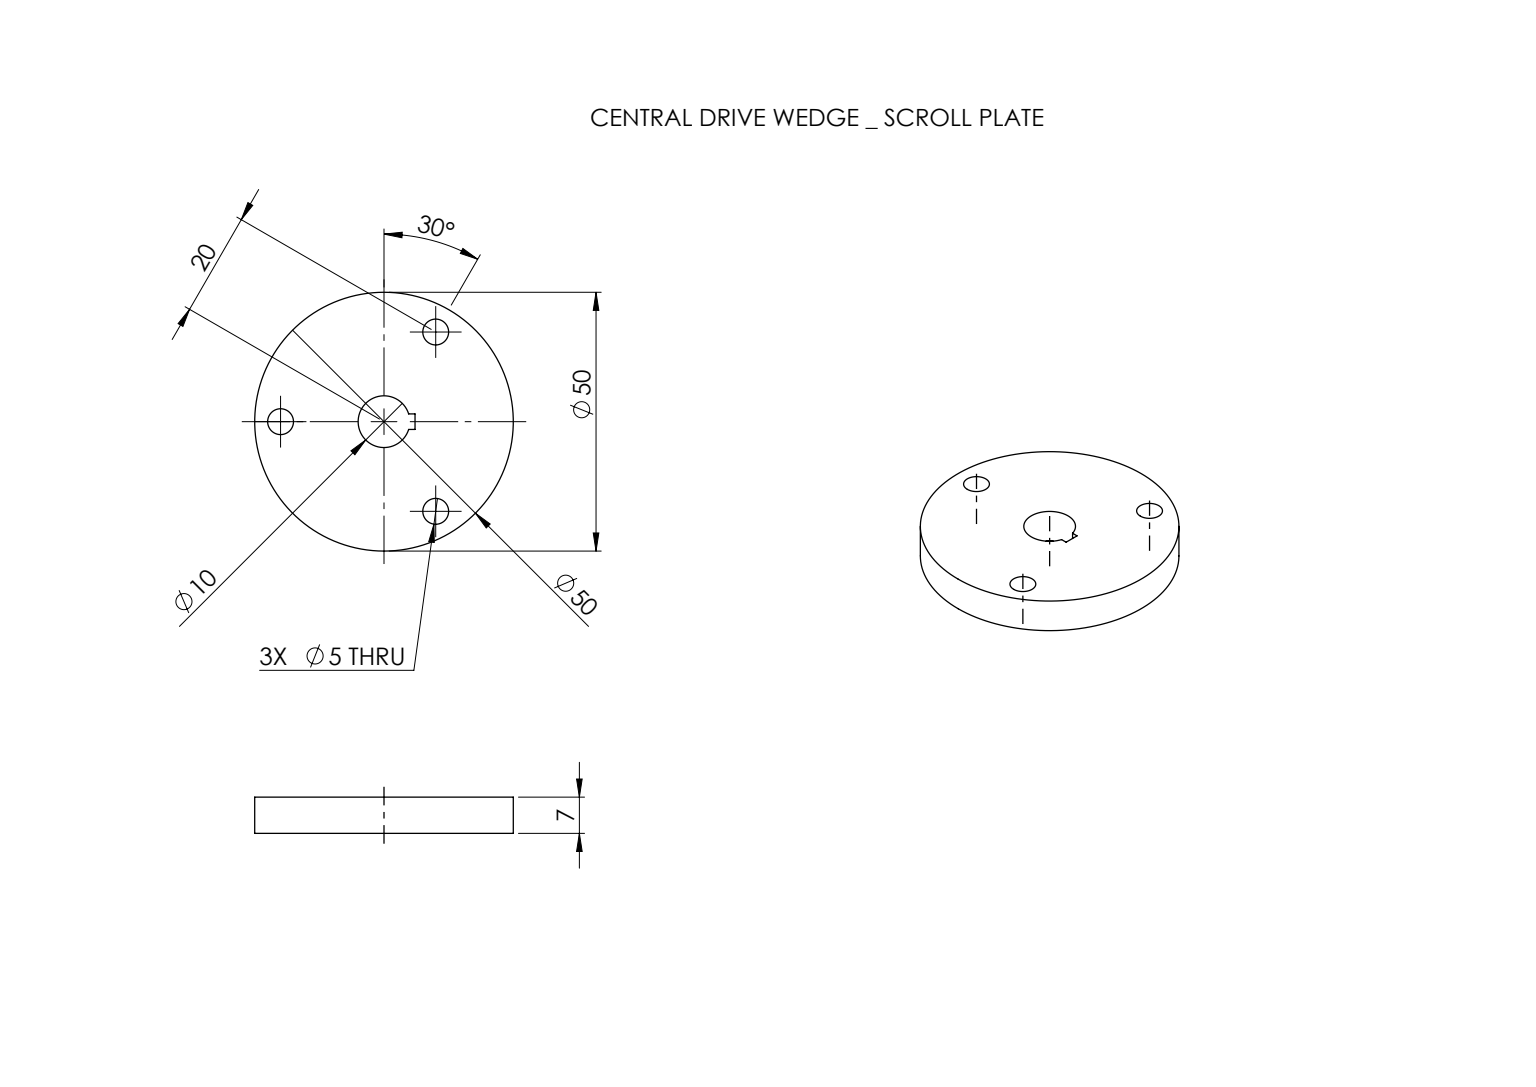
ISO-10303-21;
HEADER;
FILE_DESCRIPTION (('STEP AP214'),
    '1' );
FILE_NAME ('Central Drive Wedge _ Scroll Plate.step',
    '2026-10-08T13:56:24',
    ( '' ),
    ( '' ),
    'SwSTEP 2.0',
    'SolidWorks 2026',
    '' );
FILE_SCHEMA (( 'AUTOMOTIVE_DESIGN' ));
ENDSEC;

DATA;
#7=CARTESIAN_POINT ( 'NONE',  ( -19.99999999999956657, -20.00000000000000000, 2.500000000000877520 ) ) ;
#32=SURFACE_STYLE_USAGE ( .BOTH. , #3487 ) ;
#36=EDGE_CURVE ( 'NONE', #5349, #13611, #14887, .T. ) ;
#57=AXIS2_PLACEMENT_3D ( 'NONE', #12926, #4133, #15222 ) ;
#85=PLANE ( 'NONE',  #15054 ) ;
#94=PRESENTATION_STYLE_ASSIGNMENT (( #15940 ) ) ;
#166=EDGE_LOOP ( 'NONE', ( #524, #8301 ) ) ;
#170=CARTESIAN_POINT ( 'NONE',  ( -19.99999999999956657, -13.00000000000000178, -2.499999999999120259 ) ) ;
#196=DIRECTION ( 'NONE',  ( 0.000000000000000000, 1.000000000000000000, 0.000000000000000000 ) ) ;
#198=ORIENTED_EDGE ( 'NONE', *, *, #1877, .T. ) ;
#211=AXIS2_PLACEMENT_3D ( 'NONE', #9858, #13319, #2262 ) ;
#223=EDGE_CURVE ( 'NONE', #8492, #2510, #15229, .T. ) ;
#249=ORIENTED_EDGE ( 'NONE', *, *, #671, .F. ) ;
#255=FACE_OUTER_BOUND ( 'NONE', #7312, .T. ) ;
#286=DIRECTION ( 'NONE',  ( -0.000000000000000000, -1.000000000000000000, -0.000000000000000000 ) ) ;
#320=DIRECTION ( 'NONE',  ( 0.000000000000000000, 0.000000000000000000, 1.000000000000000000 ) ) ;
#354=CYLINDRICAL_SURFACE ( 'NONE', #57, 2.500000000000000444 ) ;
#358=CARTESIAN_POINT ( 'NONE',  ( -19.99999999999956657, -20.00000000000000000, 8.786575603324269439E-13 ) ) ;
#370=DIRECTION ( 'NONE',  ( -1.000000000000000000, 0.000000000000000000, -0.000000000000000000 ) ) ;
#437=EDGE_CURVE ( 'NONE', #15006, #14231, #6144, .T. ) ;
#524=ORIENTED_EDGE ( 'NONE', *, *, #6442, .T. ) ;
#527=CARTESIAN_POINT ( 'NONE',  ( 9.999999999999891642, -13.00000000000000178, -17.32050807568883499 ) ) ;
#606=CARTESIAN_POINT ( 'NONE',  ( 3.061616997868383043E-15, -13.00000000000000178, 25.00000000000000000 ) ) ;
#609=PRODUCT ( 'Central Drive Wedge _ Scroll Plate', 'Central Drive Wedge _ Scroll Plate', '', ( #8672 ) ) ;
#629=CARTESIAN_POINT ( 'NONE',  ( 0.000000000000000000, -13.00000000000000178, 0.000000000000000000 ) ) ;
#638=ORIENTED_EDGE ( 'NONE', *, *, #11162, .F. ) ;
#644=AXIS2_PLACEMENT_3D ( 'NONE', #5171, #10099, #12584 ) ;
#669=DIRECTION ( 'NONE',  ( 0.000000000000000000, 0.000000000000000000, 1.000000000000000000 ) ) ;
#671=EDGE_CURVE ( 'NONE', #11646, #7839, #3553, .T. ) ;
#723=APPLICATION_CONTEXT ( 'automotive_design' ) ;
#730=DIRECTION ( 'NONE',  ( 0.000000000000000000, 0.000000000000000000, -1.000000000000000000 ) ) ;
#737=DIRECTION ( 'NONE',  ( -0.000000000000000000, -1.000000000000000000, -0.000000000000000000 ) ) ;
#745=CIRCLE ( 'NONE', #4086, 2.499999999999998668 ) ;
#773=EDGE_LOOP ( 'NONE', ( #6443, #12124, #14926, #9073 ) ) ;
#853=DIRECTION ( 'NONE',  ( 0.000000000000000000, 1.000000000000000000, 0.000000000000000000 ) ) ;
#854=CIRCLE ( 'NONE', #9367, 2.499999999999998668 ) ;
#857=CARTESIAN_POINT ( 'NONE',  ( 4.769696007084728073, -20.00000000000000000, -1.500000000000000000 ) ) ;
#869=VERTEX_POINT ( 'NONE', #9235 ) ;
#918=AXIS2_PLACEMENT_3D ( 'NONE', #15837, #15765, #9600 ) ;
#928=VERTEX_POINT ( 'NONE', #6734 ) ;
#931=ORIENTED_EDGE ( 'NONE', *, *, #3922, .F. ) ;
#935=CARTESIAN_POINT ( 'NONE',  ( 0.000000000000000000, -20.00000000000000000, 0.000000000000000000 ) ) ;
#1000=DIRECTION ( 'NONE',  ( -0.000000000000000000, -1.000000000000000000, -0.000000000000000000 ) ) ;
#1016=LINE ( 'NONE', #4965, #2526 ) ;
#1021=AXIS2_PLACEMENT_3D ( 'NONE', #527, #286, #7723 ) ;
#1047=CARTESIAN_POINT ( 'NONE',  ( 6.000000000000000000, -20.00000000000000000, 1.500000000000000000 ) ) ;
#1069=EDGE_LOOP ( 'NONE', ( #13580, #15469, #3315, #3056 ) ) ;
#1076=ADVANCED_FACE ( 'NONE', ( #7046 ), #10609, .T. ) ;
#1110=CARTESIAN_POINT ( 'NONE',  ( 3.061616997868383043E-15, -20.00000000000000000, 25.00000000000000000 ) ) ;
#1136=CARTESIAN_POINT ( 'NONE',  ( 0.000000000000000000, -13.00000000000000178, 0.000000000000000000 ) ) ;
#1138=AXIS2_PLACEMENT_3D ( 'NONE', #6971, #10753, #14236 ) ;
#1205=FACE_OUTER_BOUND ( 'NONE', #4446, .T. ) ;
#1206=EDGE_CURVE ( 'NONE', #8828, #2328, #11225, .T. ) ;
#1229=CARTESIAN_POINT ( 'NONE',  ( 9.999999999999891642, -20.00000000000000000, -17.32050807568883499 ) ) ;
#1230=ORIENTED_EDGE ( 'NONE', *, *, #3922, .T. ) ;
#1251=LINE ( 'NONE', #6199, #8673 ) ;
#1260=DIRECTION ( 'NONE',  ( 0.000000000000000000, 1.000000000000000000, 0.000000000000000000 ) ) ;
#1308=DIRECTION ( 'NONE',  ( 0.000000000000000000, 1.000000000000000000, 0.000000000000000000 ) ) ;
#1313=ADVANCED_FACE ( 'NONE', ( #4853, #14711, #7357, #1205, #6151 ), #85, .F. ) ;
#1416=FACE_BOUND ( 'NONE', #3456, .T. ) ;
#1429=ORIENTED_EDGE ( 'NONE', *, *, #14917, .F. ) ;
#1493=AXIS2_PLACEMENT_3D ( 'NONE', #3815, #1630, #1554 ) ;
#1505=ORIENTED_EDGE ( 'NONE', *, *, #8244, .F. ) ;
#1554=DIRECTION ( 'NONE',  ( 0.000000000000000000, 0.000000000000000000, 1.000000000000000000 ) ) ;
#1582=PLANE ( 'NONE',  #15664 ) ;
#1630=DIRECTION ( 'NONE',  ( 0.000000000000000000, 1.000000000000000000, 0.000000000000000000 ) ) ;
#1650=CARTESIAN_POINT ( 'NONE',  ( 0.000000000000000000, -13.00000000000000178, 0.000000000000000000 ) ) ;
#1672=VERTEX_POINT ( 'NONE', #8479 ) ;
#1729=CARTESIAN_POINT ( 'NONE',  ( 3.061616997868383043E-15, -13.00000000000000178, 25.00000000000000000 ) ) ;
#1803=DIRECTION ( 'NONE',  ( -0.000000000000000000, -1.000000000000000000, -0.000000000000000000 ) ) ;
#1856=ORIENTED_EDGE ( 'NONE', *, *, #8793, .T. ) ;
#1875=EDGE_CURVE ( 'NONE', #11646, #2119, #5705, .T. ) ;
#1877=EDGE_CURVE ( 'NONE', #12259, #8828, #854, .T. ) ;
#1949=VECTOR ( 'NONE', #2580, 1000.000000000000000 ) ;
#1970=DIRECTION ( 'NONE',  ( 0.000000000000000000, 0.000000000000000000, -1.000000000000000000 ) ) ;
#2034=ORIENTED_EDGE ( 'NONE', *, *, #8902, .F. ) ;
#2093=ORIENTED_EDGE ( 'NONE', *, *, #14991, .F. ) ;
#2104=FACE_OUTER_BOUND ( 'NONE', #6226, .T. ) ;
#2119=VERTEX_POINT ( 'NONE', #12763 ) ;
#2122=DIRECTION ( 'NONE',  ( -0.000000000000000000, -1.000000000000000000, -0.000000000000000000 ) ) ;
#2170=ADVANCED_FACE ( 'NONE', ( #13821 ), #354, .F. ) ;
#2172=EDGE_CURVE ( 'NONE', #5460, #928, #5592, .T. ) ;
#2239=CARTESIAN_POINT ( 'NONE',  ( 10.00000000000098765, -13.00000000000000178, 14.82050807568871065 ) ) ;
#2246=AXIS2_PLACEMENT_3D ( 'NONE', #935, #5861, #4648 ) ;
#2262=DIRECTION ( 'NONE',  ( 0.000000000000000000, 0.000000000000000000, -1.000000000000000000 ) ) ;
#2268=SURFACE_SIDE_STYLE ('',( #7456 ) ) ;
#2277=ADVANCED_FACE ( 'NONE', ( #2104 ), #14474, .F. ) ;
#2310=ORIENTED_EDGE ( 'NONE', *, *, #11766, .T. ) ;
#2328=VERTEX_POINT ( 'NONE', #3328 ) ;
#2372=CARTESIAN_POINT ( 'NONE',  ( 6.000000000000000000, -20.00000000000000000, -1.500000000000000000 ) ) ;
#2394=ORIENTED_EDGE ( 'NONE', *, *, #9392, .F. ) ;
#2419=FACE_OUTER_BOUND ( 'NONE', #1069, .T. ) ;
#2435=CARTESIAN_POINT ( 'NONE',  ( 10.00000000000098765, -20.00000000000000000, 17.32050807568871065 ) ) ;
#2510=VERTEX_POINT ( 'NONE', #8740 ) ;
#2516=CIRCLE ( 'NONE', #8745, 5.000000000000000000 ) ;
#2526=VECTOR ( 'NONE', #10801, 1000.000000000000000 ) ;
#2564=DIRECTION ( 'NONE',  ( 1.000000000000000000, 0.000000000000000000, 0.000000000000000000 ) ) ;
#2566=CIRCLE ( 'NONE', #8025, 2.499999999999998668 ) ;
#2580=DIRECTION ( 'NONE',  ( 1.000000000000000000, 0.000000000000000000, 0.000000000000000000 ) ) ;
#2622=ORIENTED_EDGE ( 'NONE', *, *, #14803, .T. ) ;
#2678=ORIENTED_EDGE ( 'NONE', *, *, #9478, .T. ) ;
#2757=DIRECTION ( 'NONE',  ( -0.000000000000000000, -1.000000000000000000, -0.000000000000000000 ) ) ;
#2773=ADVANCED_FACE ( 'NONE', ( #10597 ), #5656, .F. ) ;
#2786=CIRCLE ( 'NONE', #6682, 2.499999999999998668 ) ;
#2867=EDGE_CURVE ( 'NONE', #15384, #5460, #10678, .T. ) ;
#2883=UNCERTAINTY_MEASURE_WITH_UNIT (LENGTH_MEASURE( 1.000000000000000082E-05 ), #13339, 'distance_accuracy_value', 'NONE');
#3001=VECTOR ( 'NONE', #9161, 1000.000000000000000 ) ;
#3018=UNCERTAINTY_MEASURE_WITH_UNIT (LENGTH_MEASURE( 1.000000000000000082E-05 ), #13477, 'distance_accuracy_value', 'NONE');
#3020=DIRECTION ( 'NONE',  ( 0.000000000000000000, 0.000000000000000000, 1.000000000000000000 ) ) ;
#3039=MECHANICAL_DESIGN_GEOMETRIC_PRESENTATION_REPRESENTATION('',(#3506),#6368);
#3053=EDGE_LOOP ( 'NONE', ( #931, #14779 ) ) ;
#3056=ORIENTED_EDGE ( 'NONE', *, *, #3832, .T. ) ;
#3077=LINE ( 'NONE', #14148, #10986 ) ;
#3180=EDGE_CURVE ( 'NONE', #15384, #3645, #14357, .T. ) ;
#3183=CARTESIAN_POINT ( 'NONE',  ( 0.000000000000000000, -20.00000000000000000, -5.000000000000000000 ) ) ;
#3186=ORIENTED_EDGE ( 'NONE', *, *, #12580, .F. ) ;
#3223=AXIS2_PLACEMENT_3D ( 'NONE', #11897, #11972, #4638 ) ;
#3277=CIRCLE ( 'NONE', #15707, 2.499999999999998668 ) ;
#3280=VECTOR ( 'NONE', #15141, 1000.000000000000000 ) ;
#3315=ORIENTED_EDGE ( 'NONE', *, *, #6324, .T. ) ;
#3328=CARTESIAN_POINT ( 'NONE',  ( -19.99999999999956657, -20.00000000000000000, -2.499999999999120259 ) ) ;
#3334=EDGE_CURVE ( 'NONE', #13329, #1672, #1016, .T. ) ;
#3396=CARTESIAN_POINT ( 'NONE',  ( 10.00000000000098765, -13.00000000000000178, 17.32050807568871065 ) ) ;
#3418=DIRECTION ( 'NONE',  ( 0.000000000000000000, 0.000000000000000000, -1.000000000000000000 ) ) ;
#3456=EDGE_LOOP ( 'NONE', ( #2394, #3186 ) ) ;
#3462=ORIENTED_EDGE ( 'NONE', *, *, #4479, .T. ) ;
#3481=CARTESIAN_POINT ( 'NONE',  ( 0.000000000000000000, -20.00000000000000000, -25.00000000000000000 ) ) ;
#3487=SURFACE_SIDE_STYLE ('',( #15953 ) ) ;
#3506=STYLED_ITEM ( 'NONE', ( #6085 ), #3780 ) ;
#3514=EDGE_LOOP ( 'NONE', ( #2034, #4762, #7178, #15022 ) ) ;
#3537=ADVANCED_FACE ( 'NONE', ( #9977 ), #14916, .F. ) ;
#3553=LINE ( 'NONE', #8513, #5240 ) ;
#3578=LINE ( 'NONE', #7381, #5890 ) ;
#3586=ORIENTED_EDGE ( 'NONE', *, *, #437, .F. ) ;
#3595=CARTESIAN_POINT ( 'NONE',  ( 6.000000000000000000, -13.00000000000000178, -1.500000000000000000 ) ) ;
#3610=EDGE_CURVE ( 'NONE', #13050, #2328, #2566, .T. ) ;
#3645=VERTEX_POINT ( 'NONE', #3183 ) ;
#3661=ORIENTED_EDGE ( 'NONE', *, *, #12894, .F. ) ;
#3707=DIRECTION ( 'NONE',  ( -0.000000000000000000, -1.000000000000000000, -0.000000000000000000 ) ) ;
#3718=FILL_AREA_STYLE ('',( #15857 ) ) ;
#3780=MANIFOLD_SOLID_BREP ( 'Cavity1', #6630 ) ;
#3815=CARTESIAN_POINT ( 'NONE',  ( 0.000000000000000000, -20.00000000000000000, 0.000000000000000000 ) ) ;
#3823=DIRECTION ( 'NONE',  ( 0.000000000000000000, 0.000000000000000000, 1.000000000000000000 ) ) ;
#3832=EDGE_CURVE ( 'NONE', #14231, #15006, #11260, .T. ) ;
#3888=DIRECTION ( 'NONE',  ( 0.000000000000000000, 0.000000000000000000, 1.000000000000000000 ) ) ;
#3899=ORIENTED_EDGE ( 'NONE', *, *, #1875, .T. ) ;
#3922=EDGE_CURVE ( 'NONE', #14864, #5642, #7921, .T. ) ;
#3986=EDGE_CURVE ( 'NONE', #8492, #8391, #4459, .T. ) ;
#4025=CARTESIAN_POINT ( 'NONE',  ( 0.000000000000000000, -20.00000000000000000, 0.000000000000000000 ) ) ;
#4043=DIRECTION ( 'NONE',  ( 0.000000000000000000, 1.000000000000000000, 0.000000000000000000 ) ) ;
#4059=CIRCLE ( 'NONE', #2246, 5.000000000000000000 ) ;
#4086=AXIS2_PLACEMENT_3D ( 'NONE', #8210, #9633, #8367 ) ;
#4125=CARTESIAN_POINT ( 'NONE',  ( 10.00000000000098765, -20.00000000000000000, 17.32050807568871065 ) ) ;
#4133=DIRECTION ( 'NONE',  ( -0.000000000000000000, -1.000000000000000000, -0.000000000000000000 ) ) ;
#4205=DIRECTION ( 'NONE',  ( 0.000000000000000000, 0.000000000000000000, 1.000000000000000000 ) ) ;
#4212=CARTESIAN_POINT ( 'NONE',  ( 6.123233995736766282E-16, -13.00000000000000178, 5.000000000000000000 ) ) ;
#4248=DIRECTION ( 'NONE',  ( 0.000000000000000000, 0.000000000000000000, 1.000000000000000000 ) ) ;
#4288=ORIENTED_EDGE ( 'NONE', *, *, #4893, .T. ) ;
#4332=DIRECTION ( 'NONE',  ( 0.000000000000000000, 1.000000000000000000, 0.000000000000000000 ) ) ;
#4446=EDGE_LOOP ( 'NONE', ( #12730, #3586 ) ) ;
#4452=DIRECTION ( 'NONE',  ( -1.000000000000000000, 0.000000000000000000, -0.000000000000000000 ) ) ;
#4454=DIRECTION ( 'NONE',  ( -0.000000000000000000, -1.000000000000000000, -0.000000000000000000 ) ) ;
#4459=LINE ( 'NONE', #12933, #3001 ) ;
#4462=( LENGTH_UNIT ( ) NAMED_UNIT ( * ) SI_UNIT ( .MILLI., .METRE. ) );
#4479=EDGE_CURVE ( 'NONE', #9721, #7795, #15171, .T. ) ;
#4618=DIRECTION ( 'NONE',  ( 0.000000000000000000, 0.000000000000000000, -1.000000000000000000 ) ) ;
#4638=DIRECTION ( 'NONE',  ( 1.000000000000000000, 0.000000000000000000, 0.000000000000000000 ) ) ;
#4648=DIRECTION ( 'NONE',  ( 0.000000000000000000, 0.000000000000000000, 1.000000000000000000 ) ) ;
#4690=LINE ( 'NONE', #13647, #12865 ) ;
#4697=( NAMED_UNIT ( * ) SI_UNIT ( $, .STERADIAN. ) SOLID_ANGLE_UNIT ( ) );
#4718=VECTOR ( 'NONE', #3707, 1000.000000000000000 ) ;
#4734=ORIENTED_EDGE ( 'NONE', *, *, #36, .F. ) ;
#4762=ORIENTED_EDGE ( 'NONE', *, *, #5244, .T. ) ;
#4775=CARTESIAN_POINT ( 'NONE',  ( 10.00000000000098765, -13.00000000000000178, 19.82050807568871065 ) ) ;
#4833=LINE ( 'NONE', #2239, #12845 ) ;
#4853=FACE_BOUND ( 'NONE', #166, .T. ) ;
#4859=VECTOR ( 'NONE', #1000, 1000.000000000000000 ) ;
#4860=DIRECTION ( 'NONE',  ( -0.000000000000000000, -1.000000000000000000, -0.000000000000000000 ) ) ;
#4863=CIRCLE ( 'NONE', #13098, 25.00000000000000000 ) ;
#4893=EDGE_CURVE ( 'NONE', #928, #8391, #4059, .T. ) ;
#4965=CARTESIAN_POINT ( 'NONE',  ( 9.999999999999891642, -13.00000000000000178, -14.82050807568883677 ) ) ;
#4970=DIRECTION ( 'NONE',  ( 0.000000000000000000, -1.000000000000000000, 0.000000000000000000 ) ) ;
#4977=DIRECTION ( 'NONE',  ( 0.000000000000000000, -0.000000000000000000, 1.000000000000000000 ) ) ;
#4982=CARTESIAN_POINT ( 'NONE',  ( 6.000000000000000000, -20.00000000000000000, 1.500000000000000000 ) ) ;
#4986=DIRECTION ( 'NONE',  ( 0.000000000000000000, 1.000000000000000000, 0.000000000000000000 ) ) ;
#5003=CARTESIAN_POINT ( 'NONE',  ( 0.000000000000000000, -20.00000000000000000, 0.000000000000000000 ) ) ;
#5171=CARTESIAN_POINT ( 'NONE',  ( -19.99999999999956657, -13.00000000000000178, 8.786575603324269439E-13 ) ) ;
#5194=DIRECTION ( 'NONE',  ( 0.000000000000000000, 0.000000000000000000, 1.000000000000000000 ) ) ;
#5240=VECTOR ( 'NONE', #7286, 1000.000000000000000 ) ;
#5244=EDGE_CURVE ( 'NONE', #6090, #15006, #5686, .T. ) ;
#5261=CARTESIAN_POINT ( 'NONE',  ( 0.000000000000000000, -13.00000000000000178, 0.000000000000000000 ) ) ;
#5301=FACE_BOUND ( 'NONE', #6982, .T. ) ;
#5314=EDGE_LOOP ( 'NONE', ( #1230, #2678, #638, #14337 ) ) ;
#5349=VERTEX_POINT ( 'NONE', #7010 ) ;
#5408=CARTESIAN_POINT ( 'NONE',  ( 0.000000000000000000, -20.00000000000000000, 1.500000000000000000 ) ) ;
#5460=VERTEX_POINT ( 'NONE', #8383 ) ;
#5461=CYLINDRICAL_SURFACE ( 'NONE', #15745, 2.499999999999998668 ) ;
#5465=DIRECTION ( 'NONE',  ( 0.000000000000000000, 0.000000000000000000, 1.000000000000000000 ) ) ;
#5470=CYLINDRICAL_SURFACE ( 'NONE', #6954, 5.000000000000000000 ) ;
#5479=CARTESIAN_POINT ( 'NONE',  ( 0.000000000000000000, -13.00000000000000178, -5.000000000000000000 ) ) ;
#5503=EDGE_CURVE ( 'NONE', #1672, #12917, #6663, .T. ) ;
#5520=ORIENTED_EDGE ( 'NONE', *, *, #3334, .T. ) ;
#5531=ORIENTED_EDGE ( 'NONE', *, *, #2172, .T. ) ;
#5573=CIRCLE ( 'NONE', #918, 2.499999999999998668 ) ;
#5592=LINE ( 'NONE', #4212, #15805 ) ;
#5599=CIRCLE ( 'NONE', #13841, 2.499999999999998668 ) ;
#5641=ORIENTED_EDGE ( 'NONE', *, *, #8244, .T. ) ;
#5642=VERTEX_POINT ( 'NONE', #4775 ) ;
#5653=ADVANCED_FACE ( 'NONE', ( #15619 ), #14637, .F. ) ;
#5656=CYLINDRICAL_SURFACE ( 'NONE', #12482, 5.000000000000000000 ) ;
#5686=LINE ( 'NONE', #606, #10526 ) ;
#5705=LINE ( 'NONE', #857, #14270 ) ;
#5714=ORIENTED_EDGE ( 'NONE', *, *, #7348, .T. ) ;
#5736=EDGE_CURVE ( 'NONE', #5642, #14864, #6143, .T. ) ;
#5857=DIRECTION ( 'NONE',  ( 0.000000000000000000, 0.000000000000000000, 1.000000000000000000 ) ) ;
#5861=DIRECTION ( 'NONE',  ( 0.000000000000000000, 1.000000000000000000, 0.000000000000000000 ) ) ;
#5890=VECTOR ( 'NONE', #12290, 1000.000000000000000 ) ;
#5919=SHAPE_REPRESENTATION_RELATIONSHIP ( 'NONE' , 'NONE' ,  #9778, #6390 ) ;
#6011=DIRECTION ( 'NONE',  ( 0.000000000000000000, 1.000000000000000000, 0.000000000000000000 ) ) ;
#6077=DIRECTION ( 'NONE',  ( 0.000000000000000000, 0.000000000000000000, -1.000000000000000000 ) ) ;
#6085=PRESENTATION_STYLE_ASSIGNMENT (( #32 ) ) ;
#6087=LINE ( 'NONE', #8369, #4859 ) ;
#6090=VERTEX_POINT ( 'NONE', #1729 ) ;
#6114=EDGE_LOOP ( 'NONE', ( #10895, #8412 ) ) ;
#6142=ORIENTED_EDGE ( 'NONE', *, *, #6676, .T. ) ;
#6143=CIRCLE ( 'NONE', #12568, 2.499999999999998668 ) ;
#6144=CIRCLE ( 'NONE', #10283, 25.00000000000000000 ) ;
#6151=FACE_BOUND ( 'NONE', #14405, .T. ) ;
#6199=CARTESIAN_POINT ( 'NONE',  ( 6.000000000000000000, -13.00000000000000178, -1.500000000000000000 ) ) ;
#6223=PRODUCT_DEFINITION ( 'UNKNOWN', '', #11789, #12546 ) ;
#6226=EDGE_LOOP ( 'NONE', ( #6424, #13535, #1856, #4734 ) ) ;
#6291=CARTESIAN_POINT ( 'NONE',  ( 0.000000000000000000, -13.00000000000000178, 0.000000000000000000 ) ) ;
#6324=EDGE_CURVE ( 'NONE', #869, #14231, #6087, .T. ) ;
#6332=ORIENTED_EDGE ( 'NONE', *, *, #15712, .T. ) ;
#6352=ORIENTED_EDGE ( 'NONE', *, *, #3986, .T. ) ;
#6356=ORIENTED_EDGE ( 'NONE', *, *, #9392, .T. ) ;
#6368=( GEOMETRIC_REPRESENTATION_CONTEXT ( 3 ) GLOBAL_UNCERTAINTY_ASSIGNED_CONTEXT ( ( #2883 ) ) GLOBAL_UNIT_ASSIGNED_CONTEXT ( ( #13339, #14808, #9803 ) ) REPRESENTATION_CONTEXT ( 'NONE', 'WORKASPACE' ) );
#6390=ADVANCED_BREP_SHAPE_REPRESENTATION ( '', ( #3780, #3223 ), #8900 ) ;
#6422=CARTESIAN_POINT ( 'NONE',  ( 0.000000000000000000, -13.00000000000000178, 1.500000000000000000 ) ) ;
#6424=ORIENTED_EDGE ( 'NONE', *, *, #9478, .F. ) ;
#6442=EDGE_CURVE ( 'NONE', #2328, #13050, #2786, .T. ) ;
#6443=ORIENTED_EDGE ( 'NONE', *, *, #12894, .T. ) ;
#6515=FACE_OUTER_BOUND ( 'NONE', #3514, .T. ) ;
#6520=FACE_BOUND ( 'NONE', #3053, .T. ) ;
#6564=MECHANICAL_DESIGN_GEOMETRIC_PRESENTATION_REPRESENTATION('',(#8382),#10938);
#6602=AXIS2_PLACEMENT_3D ( 'NONE', #4125, #10198, #13977 ) ;
#6630=CLOSED_SHELL ( 'NONE', ( #8288, #2170, #10775, #5653, #7709, #15881, #12195, #1313, #12636, #2773, #10449, #2277, #13212, #1076, #3537, #10545 ) ) ;
#6656=CARTESIAN_POINT ( 'NONE',  ( 9.999999999999891642, -20.00000000000000000, -17.32050807568883499 ) ) ;
#6663=CIRCLE ( 'NONE', #11546, 2.499999999999998668 ) ;
#6676=EDGE_CURVE ( 'NONE', #2119, #3645, #2516, .T. ) ;
#6682=AXIS2_PLACEMENT_3D ( 'NONE', #358, #1308, #8840 ) ;
#6686=ORIENTED_EDGE ( 'NONE', *, *, #1206, .T. ) ;
#6734=CARTESIAN_POINT ( 'NONE',  ( 6.123233995736766282E-16, -20.00000000000000000, 5.000000000000000000 ) ) ;
#6818=AXIS2_PLACEMENT_3D ( 'NONE', #11423, #10068, #370 ) ;
#6891=DIRECTION ( 'NONE',  ( 0.000000000000000000, 0.000000000000000000, -1.000000000000000000 ) ) ;
#6928=CARTESIAN_POINT ( 'NONE',  ( -19.99999999999956657, -13.00000000000000178, 8.786575603324269439E-13 ) ) ;
#6954=AXIS2_PLACEMENT_3D ( 'NONE', #629, #10483, #12804 ) ;
#6959=CARTESIAN_POINT ( 'NONE',  ( 4.769696007084728073, -13.00000000000000178, 1.500000000000000000 ) ) ;
#6971=CARTESIAN_POINT ( 'NONE',  ( 0.000000000000000000, -13.00000000000000178, 0.000000000000000000 ) ) ;
#6979=EDGE_LOOP ( 'NONE', ( #12956, #11485 ) ) ;
#6982=EDGE_LOOP ( 'NONE', ( #9556, #9009, #14858, #7856, #3661, #13785 ) ) ;
#7010=CARTESIAN_POINT ( 'NONE',  ( 10.00000000000098765, -20.00000000000000000, 19.82050807568871065 ) ) ;
#7029=LINE ( 'NONE', #11054, #12606 ) ;
#7046=FACE_OUTER_BOUND ( 'NONE', #10152, .T. ) ;
#7052=CARTESIAN_POINT ( 'NONE',  ( 0.000000000000000000, -13.00000000000000178, 0.000000000000000000 ) ) ;
#7178=ORIENTED_EDGE ( 'NONE', *, *, #437, .T. ) ;
#7286=DIRECTION ( 'NONE',  ( 1.000000000000000000, 0.000000000000000000, 0.000000000000000000 ) ) ;
#7312=EDGE_LOOP ( 'NONE', ( #11973, #198, #6686, #10407 ) ) ;
#7345=ORIENTED_EDGE ( 'NONE', *, *, #1206, .F. ) ;
#7348=EDGE_CURVE ( 'NONE', #2510, #7839, #7029, .T. ) ;
#7357=FACE_BOUND ( 'NONE', #6114, .T. ) ;
#7373=AXIS2_PLACEMENT_3D ( 'NONE', #8829, #11395, #4205 ) ;
#7381=CARTESIAN_POINT ( 'NONE',  ( 10.00000000000098765, -13.00000000000000178, 19.82050807568871065 ) ) ;
#7382=CIRCLE ( 'NONE', #6602, 2.499999999999998668 ) ;
#7388=DIRECTION ( 'NONE',  ( 0.000000000000000000, 1.000000000000000000, 0.000000000000000000 ) ) ;
#7450=DIRECTION ( 'NONE',  ( 0.000000000000000000, -1.000000000000000000, 0.000000000000000000 ) ) ;
#7456=SURFACE_STYLE_FILL_AREA ( #3718 ) ;
#7542=CARTESIAN_POINT ( 'NONE',  ( 9.999999999999891642, -13.00000000000000178, -17.32050807568883499 ) ) ;
#7610=COLOUR_RGB ( '', 0.31764706, 0.68627451, 0.89019608) ;
#7650=CIRCLE ( 'NONE', #1138, 5.000000000000000000 ) ;
#7681=LINE ( 'NONE', #10015, #15649 ) ;
#7709=ADVANCED_FACE ( 'NONE', ( #7904 ), #5470, .F. ) ;
#7723=DIRECTION ( 'NONE',  ( 0.000000000000000000, 0.000000000000000000, -1.000000000000000000 ) ) ;
#7769=CARTESIAN_POINT ( 'NONE',  ( 4.769696007084728073, -13.00000000000000178, -1.500000000000000000 ) ) ;
#7795=VERTEX_POINT ( 'NONE', #2372 ) ;
#7817=ORIENTED_EDGE ( 'NONE', *, *, #11164, .F. ) ;
#7822=FACE_BOUND ( 'NONE', #14814, .T. ) ;
#7839=VERTEX_POINT ( 'NONE', #3595 ) ;
#7856=ORIENTED_EDGE ( 'NONE', *, *, #2867, .F. ) ;
#7904=FACE_OUTER_BOUND ( 'NONE', #773, .T. ) ;
#7921=CIRCLE ( 'NONE', #15449, 2.499999999999998668 ) ;
#7988=DIRECTION ( 'NONE',  ( 0.000000000000000000, 1.000000000000000000, 0.000000000000000000 ) ) ;
#8021=ORIENTED_EDGE ( 'NONE', *, *, #223, .T. ) ;
#8025=AXIS2_PLACEMENT_3D ( 'NONE', #11891, #8293, #3020 ) ;
#8064=APPLICATION_CONTEXT ( 'automotive_design' ) ;
#8210=CARTESIAN_POINT ( 'NONE',  ( 9.999999999999891642, -13.00000000000000178, -17.32050807568883499 ) ) ;
#8244=EDGE_CURVE ( 'NONE', #2510, #9721, #4690, .T. ) ;
#8288=ADVANCED_FACE ( 'NONE', ( #9614 ), #8430, .F. ) ;
#8293=DIRECTION ( 'NONE',  ( 0.000000000000000000, 1.000000000000000000, 0.000000000000000000 ) ) ;
#8301=ORIENTED_EDGE ( 'NONE', *, *, #3610, .T. ) ;
#8367=DIRECTION ( 'NONE',  ( 0.000000000000000000, 0.000000000000000000, 1.000000000000000000 ) ) ;
#8369=CARTESIAN_POINT ( 'NONE',  ( 0.000000000000000000, -13.00000000000000178, -25.00000000000000000 ) ) ;
#8372=CARTESIAN_POINT ( 'NONE',  ( 9.999999999999891642, -13.00000000000000178, -17.32050807568883499 ) ) ;
#8382=STYLED_ITEM ( 'NONE', ( #94 ), #6390 ) ;
#8383=CARTESIAN_POINT ( 'NONE',  ( 6.123233995736766282E-16, -13.00000000000000178, 5.000000000000000000 ) ) ;
#8391=VERTEX_POINT ( 'NONE', #9141 ) ;
#8412=ORIENTED_EDGE ( 'NONE', *, *, #5503, .T. ) ;
#8430=CYLINDRICAL_SURFACE ( 'NONE', #211, 2.499999999999998668 ) ;
#8479=CARTESIAN_POINT ( 'NONE',  ( 9.999999999999891642, -20.00000000000000000, -14.82050807568883677 ) ) ;
#8492=VERTEX_POINT ( 'NONE', #6959 ) ;
#8513=CARTESIAN_POINT ( 'NONE',  ( 0.000000000000000000, -13.00000000000000178, -1.500000000000000000 ) ) ;
#8672=PRODUCT_CONTEXT ( 'NONE', #723, 'mechanical' ) ;
#8673=VECTOR ( 'NONE', #4970, 1000.000000000000000 ) ;
#8680=VECTOR ( 'NONE', #2564, 1000.000000000000000 ) ;
#8731=DIRECTION ( 'NONE',  ( -0.000000000000000000, -1.000000000000000000, -0.000000000000000000 ) ) ;
#8740=CARTESIAN_POINT ( 'NONE',  ( 6.000000000000000000, -13.00000000000000178, 1.500000000000000000 ) ) ;
#8745=AXIS2_PLACEMENT_3D ( 'NONE', #4025, #12500, #8893 ) ;
#8793=EDGE_CURVE ( 'NONE', #14864, #13611, #4833, .T. ) ;
#8806=FACE_OUTER_BOUND ( 'NONE', #12365, .T. ) ;
#8828=VERTEX_POINT ( 'NONE', #11291 ) ;
#8829=CARTESIAN_POINT ( 'NONE',  ( 0.000000000000000000, -20.00000000000000000, 0.000000000000000000 ) ) ;
#8840=DIRECTION ( 'NONE',  ( 0.000000000000000000, 0.000000000000000000, 1.000000000000000000 ) ) ;
#8868=DIRECTION ( 'NONE',  ( 0.000000000000000000, 1.000000000000000000, 0.000000000000000000 ) ) ;
#8893=DIRECTION ( 'NONE',  ( 0.000000000000000000, 0.000000000000000000, 1.000000000000000000 ) ) ;
#8900=( GEOMETRIC_REPRESENTATION_CONTEXT ( 3 ) GLOBAL_UNCERTAINTY_ASSIGNED_CONTEXT ( ( #14825 ) ) GLOBAL_UNIT_ASSIGNED_CONTEXT ( ( #4462, #10767, #10535 ) ) REPRESENTATION_CONTEXT ( 'NONE', 'WORKASPACE' ) );
#8902=EDGE_CURVE ( 'NONE', #6090, #869, #4863, .T. ) ;
#8947=ORIENTED_EDGE ( 'NONE', *, *, #14917, .T. ) ;
#8949=FACE_OUTER_BOUND ( 'NONE', #12491, .T. ) ;
#8972=CYLINDRICAL_SURFACE ( 'NONE', #644, 2.499999999999998668 ) ;
#8987=CARTESIAN_POINT ( 'NONE',  ( 10.00000000000098765, -13.00000000000000178, 14.82050807568871065 ) ) ;
#9009=ORIENTED_EDGE ( 'NONE', *, *, #223, .F. ) ;
#9028=ORIENTED_EDGE ( 'NONE', *, *, #5503, .F. ) ;
#9038=CARTESIAN_POINT ( 'NONE',  ( 10.00000000000098765, -20.00000000000000000, 14.82050807568871065 ) ) ;
#9073=ORIENTED_EDGE ( 'NONE', *, *, #1875, .F. ) ;
#9082=DIRECTION ( 'NONE',  ( 0.000000000000000000, 1.000000000000000000, 0.000000000000000000 ) ) ;
#9086=EDGE_LOOP ( 'NONE', ( #6356, #5520, #11999, #1429 ) ) ;
#9141=CARTESIAN_POINT ( 'NONE',  ( 4.769696007084728073, -20.00000000000000000, 1.500000000000000000 ) ) ;
#9147=ORIENTED_EDGE ( 'NONE', *, *, #2172, .F. ) ;
#9161=DIRECTION ( 'NONE',  ( 0.000000000000000000, -1.000000000000000000, 0.000000000000000000 ) ) ;
#9215=AXIS2_PLACEMENT_3D ( 'NONE', #10081, #8868, #5465 ) ;
#9233=CARTESIAN_POINT ( 'NONE',  ( 9.999999999999891642, -20.00000000000000000, -19.82050807568883499 ) ) ;
#9235=CARTESIAN_POINT ( 'NONE',  ( 0.000000000000000000, -13.00000000000000178, -25.00000000000000000 ) ) ;
#9241=AXIS2_PLACEMENT_3D ( 'NONE', #7052, #4860, #4618 ) ;
#9343=CARTESIAN_POINT ( 'NONE',  ( 0.000000000000000000, -20.00000000000000000, 0.000000000000000000 ) ) ;
#9351=DIRECTION ( 'NONE',  ( -0.000000000000000000, -1.000000000000000000, -0.000000000000000000 ) ) ;
#9367=AXIS2_PLACEMENT_3D ( 'NONE', #6928, #7988, #4248 ) ;
#9392=EDGE_CURVE ( 'NONE', #11894, #13329, #745, .T. ) ;
#9477=ORIENTED_EDGE ( 'NONE', *, *, #11766, .F. ) ;
#9478=EDGE_CURVE ( 'NONE', #5642, #5349, #3578, .T. ) ;
#9556=ORIENTED_EDGE ( 'NONE', *, *, #7348, .F. ) ;
#9600=DIRECTION ( 'NONE',  ( 0.000000000000000000, 0.000000000000000000, 1.000000000000000000 ) ) ;
#9614=FACE_OUTER_BOUND ( 'NONE', #13172, .T. ) ;
#9631=VECTOR ( 'NONE', #9351, 1000.000000000000000 ) ;
#9633=DIRECTION ( 'NONE',  ( 0.000000000000000000, 1.000000000000000000, 0.000000000000000000 ) ) ;
#9721=VERTEX_POINT ( 'NONE', #1047 ) ;
#9758=DIRECTION ( 'NONE',  ( -0.000000000000000000, -1.000000000000000000, -0.000000000000000000 ) ) ;
#9778=SHAPE_REPRESENTATION ( 'Central Drive Wedge _ Scroll Plate', ( #3223 ), #8900 ) ;
#9788=ORIENTED_EDGE ( 'NONE', *, *, #12740, .T. ) ;
#9803=( NAMED_UNIT ( * ) SI_UNIT ( $, .STERADIAN. ) SOLID_ANGLE_UNIT ( ) );
#9836=DIRECTION ( 'NONE',  ( 0.000000000000000000, 0.000000000000000000, 1.000000000000000000 ) ) ;
#9858=CARTESIAN_POINT ( 'NONE',  ( -19.99999999999956657, -13.00000000000000178, 8.786575603324269439E-13 ) ) ;
#9930=DIRECTION ( 'NONE',  ( 0.000000000000000000, 1.000000000000000000, 0.000000000000000000 ) ) ;
#9977=FACE_OUTER_BOUND ( 'NONE', #13204, .T. ) ;
#9990=CIRCLE ( 'NONE', #12040, 5.000000000000000000 ) ;
#10015=CARTESIAN_POINT ( 'NONE',  ( -19.99999999999956657, -13.00000000000000178, 2.500000000000877520 ) ) ;
#10057=ORIENTED_EDGE ( 'NONE', *, *, #4479, .F. ) ;
#10068=DIRECTION ( 'NONE',  ( 0.000000000000000000, 0.000000000000000000, -1.000000000000000000 ) ) ;
#10081=CARTESIAN_POINT ( 'NONE',  ( 0.000000000000000000, -13.00000000000000178, 0.000000000000000000 ) ) ;
#10099=DIRECTION ( 'NONE',  ( -0.000000000000000000, -1.000000000000000000, -0.000000000000000000 ) ) ;
#10130=FACE_OUTER_BOUND ( 'NONE', #9086, .T. ) ;
#10152=EDGE_LOOP ( 'NONE', ( #10057, #1505, #5714, #6332 ) ) ;
#10157=CARTESIAN_POINT ( 'NONE',  ( -19.99999999999956657, -13.00000000000000178, 2.500000000000877520 ) ) ;
#10198=DIRECTION ( 'NONE',  ( 0.000000000000000000, 1.000000000000000000, 0.000000000000000000 ) ) ;
#10215=CYLINDRICAL_SURFACE ( 'NONE', #1021, 2.499999999999998668 ) ;
#10235=CYLINDRICAL_SURFACE ( 'NONE', #10459, 25.00000000000000000 ) ;
#10255=AXIS2_PLACEMENT_3D ( 'NONE', #1136, #13483, #6077 ) ;
#10283=AXIS2_PLACEMENT_3D ( 'NONE', #9343, #4332, #5857 ) ;
#10284=EDGE_LOOP ( 'NONE', ( #13309, #5531, #7817, #15748 ) ) ;
#10407=ORIENTED_EDGE ( 'NONE', *, *, #3610, .F. ) ;
#10449=ADVANCED_FACE ( 'NONE', ( #8806 ), #5461, .F. ) ;
#10459=AXIS2_PLACEMENT_3D ( 'NONE', #1650, #13186, #1970 ) ;
#10483=DIRECTION ( 'NONE',  ( -0.000000000000000000, -1.000000000000000000, -0.000000000000000000 ) ) ;
#10526=VECTOR ( 'NONE', #1803, 1000.000000000000000 ) ;
#10535=( NAMED_UNIT ( * ) SI_UNIT ( $, .STERADIAN. ) SOLID_ANGLE_UNIT ( ) );
#10545=ADVANCED_FACE ( 'NONE', ( #11741 ), #15729, .T. ) ;
#10597=FACE_OUTER_BOUND ( 'NONE', #12953, .T. ) ;
#10603=ORIENTED_EDGE ( 'NONE', *, *, #15712, .F. ) ;
#10609=PLANE ( 'NONE',  #14266 ) ;
#10678=CIRCLE ( 'NONE', #13745, 5.000000000000000000 ) ;
#10686=EDGE_CURVE ( 'NONE', #12917, #1672, #3277, .T. ) ;
#10706=CARTESIAN_POINT ( 'NONE',  ( 0.000000000000000000, -13.00000000000000178, 1.500000000000000000 ) ) ;
#10753=DIRECTION ( 'NONE',  ( 0.000000000000000000, 1.000000000000000000, 0.000000000000000000 ) ) ;
#10755=AXIS2_PLACEMENT_3D ( 'NONE', #2435, #7388, #12295 ) ;
#10762=VECTOR ( 'NONE', #13865, 1000.000000000000000 ) ;
#10767=( NAMED_UNIT ( * ) PLANE_ANGLE_UNIT ( ) SI_UNIT ( $, .RADIAN. ) );
#10775=ADVANCED_FACE ( 'NONE', ( #10130 ), #10215, .F. ) ;
#10801=DIRECTION ( 'NONE',  ( -0.000000000000000000, -1.000000000000000000, -0.000000000000000000 ) ) ;
#10832=AXIS2_PLACEMENT_3D ( 'NONE', #10706, #15801, #12057 ) ;
#10840=CARTESIAN_POINT ( 'NONE',  ( 10.00000000000098765, -13.00000000000000178, 17.32050807568871065 ) ) ;
#10895=ORIENTED_EDGE ( 'NONE', *, *, #10686, .T. ) ;
#10938=( GEOMETRIC_REPRESENTATION_CONTEXT ( 3 ) GLOBAL_UNCERTAINTY_ASSIGNED_CONTEXT ( ( #3018 ) ) GLOBAL_UNIT_ASSIGNED_CONTEXT ( ( #13477, #13562, #4697 ) ) REPRESENTATION_CONTEXT ( 'NONE', 'WORKASPACE' ) );
#10986=VECTOR ( 'NONE', #737, 1000.000000000000000 ) ;
#11003=ORIENTED_EDGE ( 'NONE', *, *, #3334, .F. ) ;
#11054=CARTESIAN_POINT ( 'NONE',  ( 6.000000000000000000, -13.00000000000000178, 1.500000000000000000 ) ) ;
#11162=EDGE_CURVE ( 'NONE', #13611, #5349, #7382, .T. ) ;
#11164=EDGE_CURVE ( 'NONE', #3645, #928, #14338, .T. ) ;
#11225=LINE ( 'NONE', #170, #4718 ) ;
#11249=CARTESIAN_POINT ( 'NONE',  ( 10.00000000000098765, -13.00000000000000178, 17.32050807568871065 ) ) ;
#11260=CIRCLE ( 'NONE', #1493, 25.00000000000000000 ) ;
#11291=CARTESIAN_POINT ( 'NONE',  ( -19.99999999999956657, -13.00000000000000178, -2.499999999999120259 ) ) ;
#11299=COLOUR_RGB ( '', 0.31764706, 0.68627451, 0.89019608) ;
#11369=DIRECTION ( 'NONE',  ( 0.000000000000000000, 1.000000000000000000, 0.000000000000000000 ) ) ;
#11395=DIRECTION ( 'NONE',  ( 0.000000000000000000, 1.000000000000000000, 0.000000000000000000 ) ) ;
#11423=CARTESIAN_POINT ( 'NONE',  ( 0.000000000000000000, -13.00000000000000178, -1.500000000000000000 ) ) ;
#11485=ORIENTED_EDGE ( 'NONE', *, *, #36, .T. ) ;
#11546=AXIS2_PLACEMENT_3D ( 'NONE', #6656, #9082, #669 ) ;
#11631=ORIENTED_EDGE ( 'NONE', *, *, #14991, .T. ) ;
#11643=ORIENTED_EDGE ( 'NONE', *, *, #12323, .T. ) ;
#11646=VERTEX_POINT ( 'NONE', #7769 ) ;
#11673=DIRECTION ( 'NONE',  ( 0.000000000000000000, -1.000000000000000000, 0.000000000000000000 ) ) ;
#11706=EDGE_CURVE ( 'NONE', #12259, #13050, #7681, .T. ) ;
#11741=FACE_OUTER_BOUND ( 'NONE', #13456, .T. ) ;
#11766=EDGE_CURVE ( 'NONE', #8391, #9721, #12420, .T. ) ;
#11769=CARTESIAN_POINT ( 'NONE',  ( 9.999999999999891642, -13.00000000000000178, -14.82050807568883677 ) ) ;
#11774=CIRCLE ( 'NONE', #9215, 25.00000000000000000 ) ;
#11778=CARTESIAN_POINT ( 'NONE',  ( 0.000000000000000000, -13.00000000000000178, 0.000000000000000000 ) ) ;
#11789=PRODUCT_DEFINITION_FORMATION_WITH_SPECIFIED_SOURCE ( 'ANY', '', #609, .NOT_KNOWN. ) ;
#11891=CARTESIAN_POINT ( 'NONE',  ( -19.99999999999956657, -20.00000000000000000, 8.786575603324269439E-13 ) ) ;
#11894=VERTEX_POINT ( 'NONE', #14041 ) ;
#11897=CARTESIAN_POINT ( 'NONE',  ( 0.000000000000000000, 0.000000000000000000, 0.000000000000000000 ) ) ;
#11939=ORIENTED_EDGE ( 'NONE', *, *, #11706, .T. ) ;
#11972=DIRECTION ( 'NONE',  ( 0.000000000000000000, 0.000000000000000000, 1.000000000000000000 ) ) ;
#11973=ORIENTED_EDGE ( 'NONE', *, *, #11706, .F. ) ;
#11999=ORIENTED_EDGE ( 'NONE', *, *, #10686, .F. ) ;
#12040=AXIS2_PLACEMENT_3D ( 'NONE', #5261, #4043, #3888 ) ;
#12057=DIRECTION ( 'NONE',  ( -1.000000000000000000, 0.000000000000000000, -0.000000000000000000 ) ) ;
#12079=ORIENTED_EDGE ( 'NONE', *, *, #6442, .F. ) ;
#12124=ORIENTED_EDGE ( 'NONE', *, *, #3180, .T. ) ;
#12154=ORIENTED_EDGE ( 'NONE', *, *, #11164, .T. ) ;
#12190=DIRECTION ( 'NONE',  ( 0.000000000000000000, 0.000000000000000000, 1.000000000000000000 ) ) ;
#12195=ADVANCED_FACE ( 'NONE', ( #7822, #1416, #8949, #6520, #5301 ), #1582, .T. ) ;
#12199=CYLINDRICAL_SURFACE ( 'NONE', #10255, 25.00000000000000000 ) ;
#12259=VERTEX_POINT ( 'NONE', #10157 ) ;
#12281=DIRECTION ( 'NONE',  ( 0.000000000000000000, 0.000000000000000000, 1.000000000000000000 ) ) ;
#12290=DIRECTION ( 'NONE',  ( -0.000000000000000000, -1.000000000000000000, -0.000000000000000000 ) ) ;
#12295=DIRECTION ( 'NONE',  ( 0.000000000000000000, 0.000000000000000000, 1.000000000000000000 ) ) ;
#12323=EDGE_CURVE ( 'NONE', #869, #6090, #11774, .T. ) ;
#12360=CARTESIAN_POINT ( 'NONE',  ( 0.000000000000000000, -20.00000000000000000, -1.500000000000000000 ) ) ;
#12365=EDGE_LOOP ( 'NONE', ( #11003, #12450, #8947, #9028 ) ) ;
#12420=LINE ( 'NONE', #5408, #8680 ) ;
#12450=ORIENTED_EDGE ( 'NONE', *, *, #12580, .T. ) ;
#12482=AXIS2_PLACEMENT_3D ( 'NONE', #11778, #13151, #730 ) ;
#12491=EDGE_LOOP ( 'NONE', ( #11643, #12858 ) ) ;
#12500=DIRECTION ( 'NONE',  ( 0.000000000000000000, 1.000000000000000000, 0.000000000000000000 ) ) ;
#12546=PRODUCT_DEFINITION_CONTEXT ( 'detailed design', #8064, 'design' ) ;
#12568=AXIS2_PLACEMENT_3D ( 'NONE', #10840, #14719, #12190 ) ;
#12580=EDGE_CURVE ( 'NONE', #13329, #11894, #5599, .T. ) ;
#12584=DIRECTION ( 'NONE',  ( 0.000000000000000000, 0.000000000000000000, -1.000000000000000000 ) ) ;
#12606=VECTOR ( 'NONE', #14691, 1000.000000000000000 ) ;
#12617=ORIENTED_EDGE ( 'NONE', *, *, #14803, .F. ) ;
#12636=ADVANCED_FACE ( 'NONE', ( #2419 ), #12199, .T. ) ;
#12730=ORIENTED_EDGE ( 'NONE', *, *, #3832, .F. ) ;
#12740=EDGE_CURVE ( 'NONE', #5460, #8492, #9990, .T. ) ;
#12763=CARTESIAN_POINT ( 'NONE',  ( 4.769696007084728073, -20.00000000000000000, -1.500000000000000000 ) ) ;
#12804=DIRECTION ( 'NONE',  ( 0.000000000000000000, 0.000000000000000000, -1.000000000000000000 ) ) ;
#12845=VECTOR ( 'NONE', #9758, 1000.000000000000000 ) ;
#12846=PRODUCT_DEFINITION_SHAPE ( 'NONE', 'NONE',  #6223 ) ;
#12858=ORIENTED_EDGE ( 'NONE', *, *, #8902, .T. ) ;
#12865=VECTOR ( 'NONE', #7450, 1000.000000000000000 ) ;
#12894=EDGE_CURVE ( 'NONE', #11646, #15384, #7650, .T. ) ;
#12917=VERTEX_POINT ( 'NONE', #9233 ) ;
#12926=CARTESIAN_POINT ( 'NONE',  ( 10.00000000000098765, -13.00000000000000178, 17.32050807568871065 ) ) ;
#12933=CARTESIAN_POINT ( 'NONE',  ( 4.769696007084728073, -20.00000000000000000, 1.500000000000000000 ) ) ;
#12953=EDGE_LOOP ( 'NONE', ( #9147, #9788, #6352, #13936 ) ) ;
#12956=ORIENTED_EDGE ( 'NONE', *, *, #11162, .T. ) ;
#13050=VERTEX_POINT ( 'NONE', #7 ) ;
#13098=AXIS2_PLACEMENT_3D ( 'NONE', #13781, #11369, #320 ) ;
#13151=DIRECTION ( 'NONE',  ( -0.000000000000000000, -1.000000000000000000, -0.000000000000000000 ) ) ;
#13166=DIRECTION ( 'NONE',  ( -0.000000000000000000, 0.000000000000000000, 1.000000000000000000 ) ) ;
#13172=EDGE_LOOP ( 'NONE', ( #11631, #11939, #12079, #7345 ) ) ;
#13186=DIRECTION ( 'NONE',  ( -0.000000000000000000, -1.000000000000000000, -0.000000000000000000 ) ) ;
#13204=EDGE_LOOP ( 'NONE', ( #3899, #2622, #10603, #249 ) ) ;
#13212=ADVANCED_FACE ( 'NONE', ( #255 ), #8972, .F. ) ;
#13309=ORIENTED_EDGE ( 'NONE', *, *, #2867, .T. ) ;
#13319=DIRECTION ( 'NONE',  ( -0.000000000000000000, -1.000000000000000000, -0.000000000000000000 ) ) ;
#13329=VERTEX_POINT ( 'NONE', #11769 ) ;
#13339=( LENGTH_UNIT ( ) NAMED_UNIT ( * ) SI_UNIT ( .MILLI., .METRE. ) );
#13456=EDGE_LOOP ( 'NONE', ( #8021, #5641, #9477, #15371 ) ) ;
#13477=( LENGTH_UNIT ( ) NAMED_UNIT ( * ) SI_UNIT ( .MILLI., .METRE. ) );
#13483=DIRECTION ( 'NONE',  ( -0.000000000000000000, -1.000000000000000000, -0.000000000000000000 ) ) ;
#13535=ORIENTED_EDGE ( 'NONE', *, *, #5736, .T. ) ;
#13562=( NAMED_UNIT ( * ) PLANE_ANGLE_UNIT ( ) SI_UNIT ( $, .RADIAN. ) );
#13580=ORIENTED_EDGE ( 'NONE', *, *, #5244, .F. ) ;
#13611=VERTEX_POINT ( 'NONE', #9038 ) ;
#13647=CARTESIAN_POINT ( 'NONE',  ( 6.000000000000000000, -13.00000000000000178, 1.500000000000000000 ) ) ;
#13726=LINE ( 'NONE', #12360, #1949 ) ;
#13745=AXIS2_PLACEMENT_3D ( 'NONE', #6291, #4986, #9836 ) ;
#13781=CARTESIAN_POINT ( 'NONE',  ( 0.000000000000000000, -13.00000000000000178, 0.000000000000000000 ) ) ;
#13785=ORIENTED_EDGE ( 'NONE', *, *, #671, .T. ) ;
#13821=FACE_OUTER_BOUND ( 'NONE', #5314, .T. ) ;
#13841=AXIS2_PLACEMENT_3D ( 'NONE', #7542, #853, #12281 ) ;
#13865=DIRECTION ( 'NONE',  ( 0.000000000000000000, 0.000000000000000000, -1.000000000000000000 ) ) ;
#13936=ORIENTED_EDGE ( 'NONE', *, *, #4893, .F. ) ;
#13977=DIRECTION ( 'NONE',  ( 0.000000000000000000, 0.000000000000000000, 1.000000000000000000 ) ) ;
#14041=CARTESIAN_POINT ( 'NONE',  ( 9.999999999999891642, -13.00000000000000178, -19.82050807568883499 ) ) ;
#14148=CARTESIAN_POINT ( 'NONE',  ( 9.999999999999891642, -13.00000000000000178, -19.82050807568883499 ) ) ;
#14231=VERTEX_POINT ( 'NONE', #3481 ) ;
#14236=DIRECTION ( 'NONE',  ( 0.000000000000000000, 0.000000000000000000, 1.000000000000000000 ) ) ;
#14266=AXIS2_PLACEMENT_3D ( 'NONE', #15537, #4452, #13166 ) ;
#14270=VECTOR ( 'NONE', #11673, 1000.000000000000000 ) ;
#14337=ORIENTED_EDGE ( 'NONE', *, *, #8793, .F. ) ;
#14338=CIRCLE ( 'NONE', #7373, 5.000000000000000000 ) ;
#14357=LINE ( 'NONE', #14439, #9631 ) ;
#14405=EDGE_LOOP ( 'NONE', ( #12617, #6142, #12154, #4288, #2310, #3462 ) ) ;
#14439=CARTESIAN_POINT ( 'NONE',  ( 0.000000000000000000, -13.00000000000000178, -5.000000000000000000 ) ) ;
#14474=CYLINDRICAL_SURFACE ( 'NONE', #15292, 2.500000000000000444 ) ;
#14565=FILL_AREA_STYLE ('',( #14731 ) ) ;
#14637=CYLINDRICAL_SURFACE ( 'NONE', #9241, 5.000000000000000000 ) ;
#14691=DIRECTION ( 'NONE',  ( 0.000000000000000000, 0.000000000000000000, -1.000000000000000000 ) ) ;
#14711=FACE_BOUND ( 'NONE', #6979, .T. ) ;
#14719=DIRECTION ( 'NONE',  ( 0.000000000000000000, 1.000000000000000000, 0.000000000000000000 ) ) ;
#14731=FILL_AREA_STYLE_COLOUR ( '', #11299 ) ;
#14779=ORIENTED_EDGE ( 'NONE', *, *, #5736, .F. ) ;
#14803=EDGE_CURVE ( 'NONE', #2119, #7795, #13726, .T. ) ;
#14806=SHAPE_DEFINITION_REPRESENTATION ( #12846, #9778 ) ;
#14808=( NAMED_UNIT ( * ) PLANE_ANGLE_UNIT ( ) SI_UNIT ( $, .RADIAN. ) );
#14814=EDGE_LOOP ( 'NONE', ( #2093, #15048 ) ) ;
#14825=UNCERTAINTY_MEASURE_WITH_UNIT (LENGTH_MEASURE( 1.000000000000000082E-05 ), #4462, 'distance_accuracy_value', 'NONE');
#14842=CARTESIAN_POINT ( 'NONE',  ( 0.000000000000000000, -13.00000000000000178, 0.000000000000000000 ) ) ;
#14858=ORIENTED_EDGE ( 'NONE', *, *, #12740, .F. ) ;
#14864=VERTEX_POINT ( 'NONE', #8987 ) ;
#14869=DIRECTION ( 'NONE',  ( 0.000000000000000000, -0.000000000000000000, 1.000000000000000000 ) ) ;
#14887=CIRCLE ( 'NONE', #10755, 2.499999999999998668 ) ;
#14916=PLANE ( 'NONE',  #6818 ) ;
#14917=EDGE_CURVE ( 'NONE', #11894, #12917, #3077, .T. ) ;
#14926=ORIENTED_EDGE ( 'NONE', *, *, #6676, .F. ) ;
#14991=EDGE_CURVE ( 'NONE', #8828, #12259, #5573, .T. ) ;
#15006=VERTEX_POINT ( 'NONE', #1110 ) ;
#15022=ORIENTED_EDGE ( 'NONE', *, *, #6324, .F. ) ;
#15048=ORIENTED_EDGE ( 'NONE', *, *, #1877, .F. ) ;
#15054=AXIS2_PLACEMENT_3D ( 'NONE', #5003, #9930, #14869 ) ;
#15141=DIRECTION ( 'NONE',  ( 1.000000000000000000, 0.000000000000000000, 0.000000000000000000 ) ) ;
#15171=LINE ( 'NONE', #4982, #10762 ) ;
#15222=DIRECTION ( 'NONE',  ( 0.000000000000000000, 0.000000000000000000, -1.000000000000000000 ) ) ;
#15229=LINE ( 'NONE', #6422, #3280 ) ;
#15292=AXIS2_PLACEMENT_3D ( 'NONE', #3396, #4454, #6891 ) ;
#15371=ORIENTED_EDGE ( 'NONE', *, *, #3986, .F. ) ;
#15384=VERTEX_POINT ( 'NONE', #5479 ) ;
#15449=AXIS2_PLACEMENT_3D ( 'NONE', #11249, #196, #5194 ) ;
#15469=ORIENTED_EDGE ( 'NONE', *, *, #12323, .F. ) ;
#15537=CARTESIAN_POINT ( 'NONE',  ( 6.000000000000000000, -13.00000000000000178, 1.500000000000000000 ) ) ;
#15619=FACE_OUTER_BOUND ( 'NONE', #10284, .T. ) ;
#15649=VECTOR ( 'NONE', #8731, 1000.000000000000000 ) ;
#15664=AXIS2_PLACEMENT_3D ( 'NONE', #14842, #1260, #4977 ) ;
#15707=AXIS2_PLACEMENT_3D ( 'NONE', #1229, #6011, #3823 ) ;
#15712=EDGE_CURVE ( 'NONE', #7839, #7795, #1251, .T. ) ;
#15729=PLANE ( 'NONE',  #10832 ) ;
#15745=AXIS2_PLACEMENT_3D ( 'NONE', #8372, #2122, #3418 ) ;
#15748=ORIENTED_EDGE ( 'NONE', *, *, #3180, .F. ) ;
#15765=DIRECTION ( 'NONE',  ( 0.000000000000000000, 1.000000000000000000, 0.000000000000000000 ) ) ;
#15801=DIRECTION ( 'NONE',  ( 0.000000000000000000, 0.000000000000000000, -1.000000000000000000 ) ) ;
#15805=VECTOR ( 'NONE', #2757, 1000.000000000000000 ) ;
#15837=CARTESIAN_POINT ( 'NONE',  ( -19.99999999999956657, -13.00000000000000178, 8.786575603324269439E-13 ) ) ;
#15857=FILL_AREA_STYLE_COLOUR ( '', #7610 ) ;
#15881=ADVANCED_FACE ( 'NONE', ( #6515 ), #10235, .T. ) ;
#15940=SURFACE_STYLE_USAGE ( .BOTH. , #2268 ) ;
#15953=SURFACE_STYLE_FILL_AREA ( #14565 ) ;
ENDSEC;
END-ISO-10303-21;
